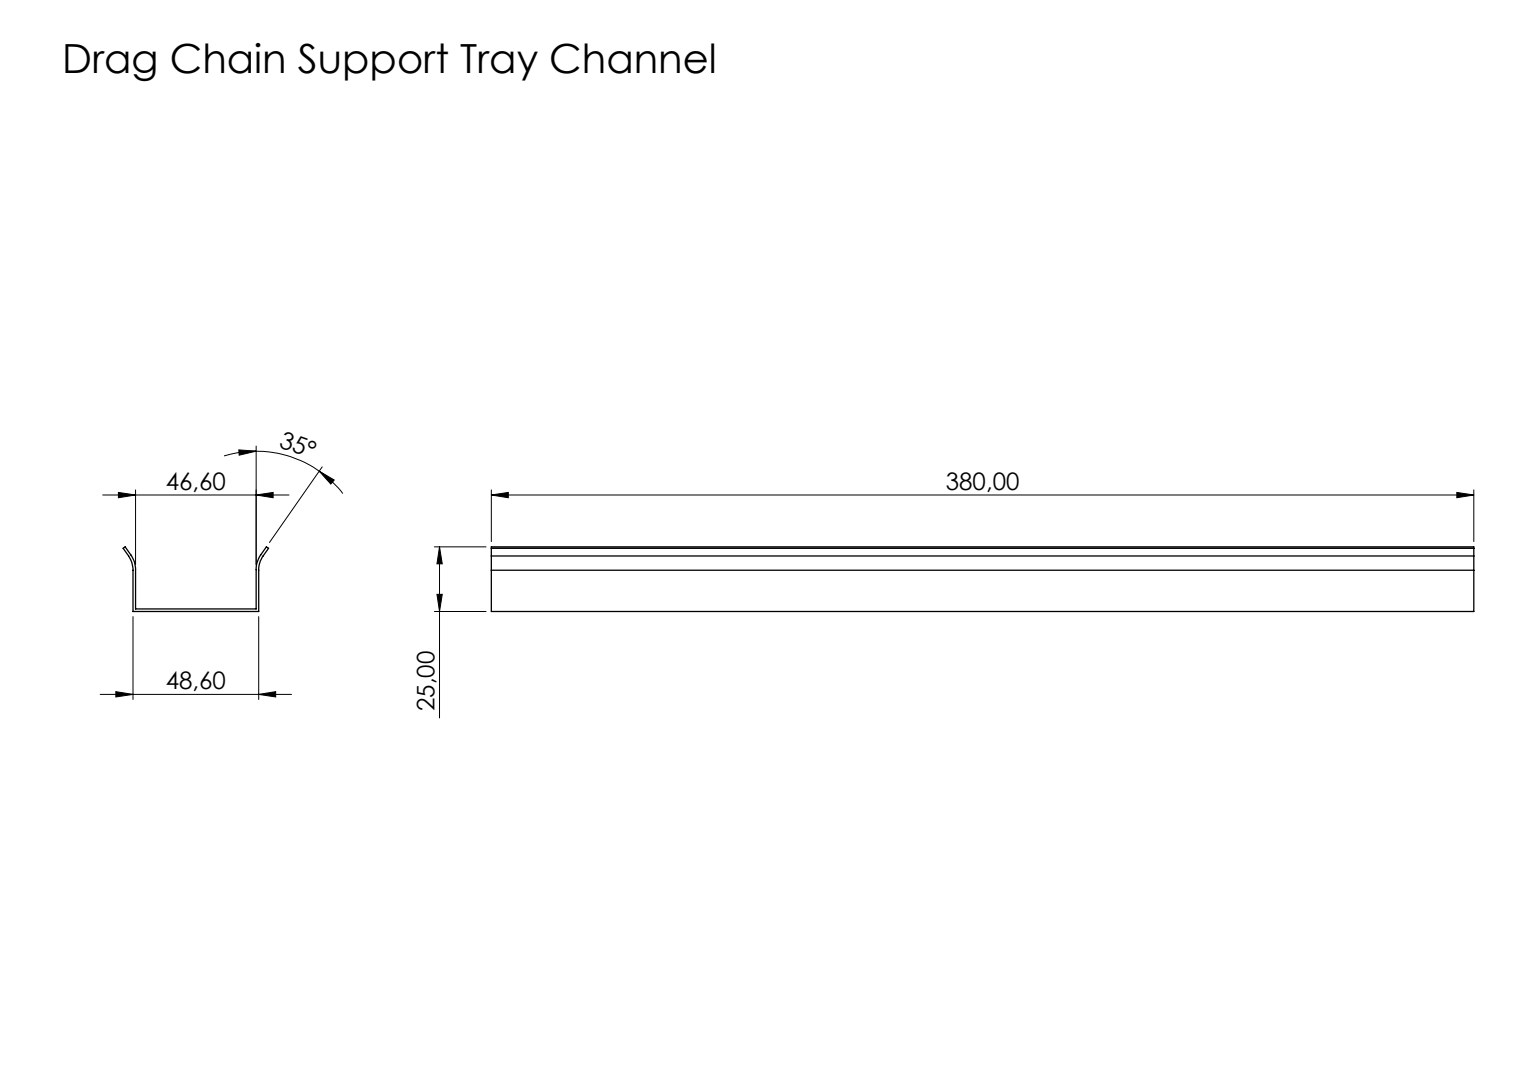
ISO-10303-21;
HEADER;
FILE_DESCRIPTION (('STEP AP214'),
    '1' );
FILE_NAME ('Drag Chain Support Tray Channel.step',
    '2026-10-08T22:59:04',
    ( '' ),
    ( '' ),
    'SwSTEP 2.0',
    'SolidWorks 2020',
    '' );
FILE_SCHEMA (( 'AUTOMOTIVE_DESIGN' ));
ENDSEC;

DATA;
#73=CARTESIAN_POINT ( 'NONE',  ( 33.30000000000001137, 3.332938107839120701, 33.00000000000000000 ) ) ;
#738=FACE_OUTER_BOUND ( 'NONE', #224116, .T. ) ;
#922=APPLICATION_CONTEXT ( 'automotive_design' ) ;
#1036=ORIENTED_EDGE ( 'NONE', *, *, #252988, .T. ) ;
#2425=AXIS2_PLACEMENT_3D ( 'NONE', #153513, #135160, #16531 ) ;
#2767=LINE ( 'NONE', #5320, #211110 ) ;
#3053=EDGE_CURVE ( 'NONE', #170483, #36666, #227559, .T. ) ;
#3540=CARTESIAN_POINT ( 'NONE',  ( 24.30000000000000071, 3.175288713399624818, -347.0000000000001137 ) ) ;
#4159=DIRECTION ( 'NONE',  ( 0.000000000000000000, 0.000000000000000000, 1.000000000000000000 ) ) ;
#4565=VECTOR ( 'NONE', #97094, 999.9999999999998863 ) ;
#4618=LINE ( 'NONE', #163716, #49347 ) ;
#4703=AXIS2_PLACEMENT_3D ( 'NONE', #177790, #57793, #79908 ) ;
#5320=CARTESIAN_POINT ( 'NONE',  ( 28.12018973533754362, 11.62642356364896123, 33.00000000000000000 ) ) ;
#5336=CIRCLE ( 'NONE', #192815, 9.500000000000001776 ) ;
#5403=ORIENTED_EDGE ( 'NONE', *, *, #105661, .F. ) ;
#5597=VERTEX_POINT ( 'NONE', #205200 ) ;
#5837=AXIS2_PLACEMENT_3D ( 'NONE', #3540, #257818, #144314 ) ;
#5882=LINE ( 'NONE', #127130, #156042 ) ;
#6762=EDGE_CURVE ( 'NONE', #161541, #211804, #135194, .T. ) ;
#6787=AXIS2_PLACEMENT_3D ( 'NONE', #52394, #130658, #31601 ) ;
#6946=ORIENTED_EDGE ( 'NONE', *, *, #257321, .T. ) ;
#7916=FACE_OUTER_BOUND ( 'NONE', #129895, .T. ) ;
#8087=ORIENTED_EDGE ( 'NONE', *, *, #57923, .T. ) ;
#8445=DIRECTION ( 'NONE',  ( 0.8191520442889919096, -0.5735764363510460484, 0.000000000000000000 ) ) ;
#9694=ORIENTED_EDGE ( 'NONE', *, *, #126812, .T. ) ;
#11133=DIRECTION ( 'NONE',  ( 1.000000000000000000, 0.000000000000000000, 0.000000000000000000 ) ) ;
#11208=ADVANCED_FACE ( 'NONE', ( #78803 ), #179241, .F. ) ;
#11741=AXIS2_PLACEMENT_3D ( 'NONE', #168935, #248426, #189738 ) ;
#13839=ADVANCED_BREP_SHAPE_REPRESENTATION ( '', ( #193773, #2425 ), #147622 ) ;
#14104=ORIENTED_EDGE ( 'NONE', *, *, #134158, .T. ) ;
#14595=PLANE ( 'NONE',  #6787 ) ;
#16293=CARTESIAN_POINT ( 'NONE',  ( 24.30000000000000071, -12.79999999999999716, -347.0000000000001137 ) ) ;
#16531=DIRECTION ( 'NONE',  ( 1.000000000000000000, 0.000000000000000000, 0.000000000000000000 ) ) ;
#16973=CARTESIAN_POINT ( 'NONE',  ( -27.30103769104855971, 12.19999999999999574, -347.0000000000001137 ) ) ;
#17586=CARTESIAN_POINT ( 'NONE',  ( -27.30103769104855971, 12.19999999999999574, 33.00000000000000000 ) ) ;
#17889=CARTESIAN_POINT ( 'NONE',  ( -24.30000000000000071, 3.175288713399619045, 33.00000000000000000 ) ) ;
#18117=DIRECTION ( 'NONE',  ( 0.5735764363510460484, -0.8191520442889919096, 0.000000000000000000 ) ) ;
#18168=DIRECTION ( 'NONE',  ( 1.070816960479510500E-16, -1.000000000000000000, 0.000000000000000000 ) ) ;
#18849=CARTESIAN_POINT ( 'NONE',  ( 33.30000000000001137, 3.332938107839120701, 33.00000000000000000 ) ) ;
#19405=ORIENTED_EDGE ( 'NONE', *, *, #195711, .T. ) ;
#19702=PLANE ( 'NONE',  #213240 ) ;
#19758=DIRECTION ( 'NONE',  ( -1.000000000000000000, 0.000000000000000000, 0.000000000000000000 ) ) ;
#20570=PLANE ( 'NONE',  #5837 ) ;
#20732=EDGE_LOOP ( 'NONE', ( #78906, #26119, #97741, #47134 ) ) ;
#20927=DIRECTION ( 'NONE',  ( -1.000000000000000000, 0.000000000000000000, 0.000000000000000000 ) ) ;
#21145=EDGE_CURVE ( 'NONE', #21183, #211804, #162402, .T. ) ;
#21183=VERTEX_POINT ( 'NONE', #80239 ) ;
#21763=ORIENTED_EDGE ( 'NONE', *, *, #207928, .T. ) ;
#21791=EDGE_CURVE ( 'NONE', #129045, #52293, #190662, .T. ) ;
#22213=VECTOR ( 'NONE', #257517, 1000.000000000000000 ) ;
#22259=CARTESIAN_POINT ( 'NONE',  ( 24.30000000000000071, 3.175288713399624818, 33.00000000000000000 ) ) ;
#22351=CARTESIAN_POINT ( 'NONE',  ( -24.30000000000000071, 3.175288713399619045, -347.0000000000001137 ) ) ;
#22631=LINE ( 'NONE', #102112, #93911 ) ;
#23564=ORIENTED_EDGE ( 'NONE', *, *, #151707, .T. ) ;
#23567=DIRECTION ( 'NONE',  ( -0.000000000000000000, 1.000000000000000000, -0.000000000000000000 ) ) ;
#23597=CARTESIAN_POINT ( 'NONE',  ( -33.80000000000000426, 3.175288713399618601, -347.0000000000001137 ) ) ;
#23706=( LENGTH_UNIT ( ) NAMED_UNIT ( * ) SI_UNIT ( .MILLI., .METRE. ) );
#24444=CLOSED_SHELL ( 'NONE', ( #93514, #231899, #33585, #223638, #74734, #90628, #232417, #255096, #257586, #97914, #165410, #200576, #127157, #116588, #142229, #84628, #136428, #11208 ) ) ;
#25351=EDGE_CURVE ( 'NONE', #161541, #81489, #168111, .T. ) ;
#25723=APPLICATION_CONTEXT ( 'automotive_design' ) ;
#26119=ORIENTED_EDGE ( 'NONE', *, *, #173029, .F. ) ;
#26230=VERTEX_POINT ( 'NONE', #239541 ) ;
#26815=( LENGTH_UNIT ( ) NAMED_UNIT ( * ) SI_UNIT ( .MILLI., .METRE. ) );
#26974=SHAPE_REPRESENTATION ( 'Drag Chain Support Tray Channel', ( #2425 ), #147622 ) ;
#27239=ORIENTED_EDGE ( 'NONE', *, *, #127036, .T. ) ;
#28179=ORIENTED_EDGE ( 'NONE', *, *, #162458, .F. ) ;
#28703=ORIENTED_EDGE ( 'NONE', *, *, #230771, .T. ) ;
#28742=VECTOR ( 'NONE', #138929, 1000.000000000000000 ) ;
#28860=VERTEX_POINT ( 'NONE', #101014 ) ;
#29155=ORIENTED_EDGE ( 'NONE', *, *, #182694, .T. ) ;
#29427=( GEOMETRIC_REPRESENTATION_CONTEXT ( 3 ) GLOBAL_UNCERTAINTY_ASSIGNED_CONTEXT ( ( #47787 ) ) GLOBAL_UNIT_ASSIGNED_CONTEXT ( ( #23706, #79762, #159350 ) ) REPRESENTATION_CONTEXT ( 'NONE', 'WORKASPACE' ) );
#29963=VECTOR ( 'NONE', #214620, 1000.000000000000000 ) ;
#30285=CARTESIAN_POINT ( 'NONE',  ( -24.30000000000000071, -12.80000000000000249, 33.00000000000000000 ) ) ;
#30300=ORIENTED_EDGE ( 'NONE', *, *, #3053, .T. ) ;
#30661=FILL_AREA_STYLE_COLOUR ( '', #135708 ) ;
#30927=ORIENTED_EDGE ( 'NONE', *, *, #130588, .T. ) ;
#31601=DIRECTION ( 'NONE',  ( -1.000000000000000000, -1.116774769942150098E-16, 0.000000000000000000 ) ) ;
#31615=ORIENTED_EDGE ( 'NONE', *, *, #154307, .F. ) ;
#31650=DIRECTION ( 'NONE',  ( -0.8191520442889914655, 0.5735764363510466035, 0.000000000000000000 ) ) ;
#32019=AXIS2_PLACEMENT_3D ( 'NONE', #73643, #131013, #153189 ) ;
#32279=CARTESIAN_POINT ( 'NONE',  ( 23.30000000000000426, 3.332938107839120701, 33.00000000000000000 ) ) ;
#32646=EDGE_CURVE ( 'NONE', #58739, #220374, #149831, .T. ) ;
#32834=ORIENTED_EDGE ( 'NONE', *, *, #151707, .F. ) ;
#33530=STYLED_ITEM ( 'NONE', ( #199767 ), #193773 ) ;
#33585=ADVANCED_FACE ( 'NONE', ( #196977 ), #256914, .T. ) ;
#34708=LINE ( 'NONE', #235434, #22213 ) ;
#34764=EDGE_CURVE ( 'NONE', #28860, #179923, #4618, .T. ) ;
#34785=DIRECTION ( 'NONE',  ( -0.000000000000000000, -0.000000000000000000, -1.000000000000000000 ) ) ;
#36258=ORIENTED_EDGE ( 'NONE', *, *, #252988, .F. ) ;
#36666=VERTEX_POINT ( 'NONE', #224393 ) ;
#36717=VECTOR ( 'NONE', #251880, 1000.000000000000000 ) ;
#37418=DIRECTION ( 'NONE',  ( 0.000000000000000000, 0.000000000000000000, 1.000000000000000000 ) ) ;
#38131=CARTESIAN_POINT ( 'NONE',  ( -24.30000000000000071, 3.175288713399619933, -347.0000000000001137 ) ) ;
#38192=EDGE_CURVE ( 'NONE', #81489, #129962, #210850, .T. ) ;
#39279=CARTESIAN_POINT ( 'NONE',  ( -27.30103769104855971, 12.19999999999999574, -347.0000000000001137 ) ) ;
#40331=DIRECTION ( 'NONE',  ( 0.000000000000000000, 0.000000000000000000, 1.000000000000000000 ) ) ;
#40973=VERTEX_POINT ( 'NONE', #97492 ) ;
#41222=VECTOR ( 'NONE', #168357, 999.9999999999998863 ) ;
#41767=LINE ( 'NONE', #121321, #217642 ) ;
#42076=VECTOR ( 'NONE', #167900, 1000.000000000000000 ) ;
#42249=VECTOR ( 'NONE', #96464, 1000.000000000000000 ) ;
#43561=CARTESIAN_POINT ( 'NONE',  ( -25.10847955711009760, 9.068702471349583405, 33.00000000000000000 ) ) ;
#44072=CARTESIAN_POINT ( 'NONE',  ( -27.30103769104855971, 12.19999999999999574, 33.00000000000000000 ) ) ;
#45239=DIRECTION ( 'NONE',  ( -0.5735764363510466035, 0.8191520442889914655, 0.000000000000000000 ) ) ;
#45827=DIRECTION ( 'NONE',  ( 0.000000000000000000, 1.000000000000000000, 0.000000000000000000 ) ) ;
#46873=VERTEX_POINT ( 'NONE', #193707 ) ;
#47134=ORIENTED_EDGE ( 'NONE', *, *, #188159, .T. ) ;
#47545=LINE ( 'NONE', #84070, #225389 ) ;
#47787=UNCERTAINTY_MEASURE_WITH_UNIT (LENGTH_MEASURE( 1.000000000000000082E-05 ), #23706, 'distance_accuracy_value', 'NONE');
#47845=ORIENTED_EDGE ( 'NONE', *, *, #137375, .T. ) ;
#48528=ORIENTED_EDGE ( 'NONE', *, *, #38192, .T. ) ;
#48882=EDGE_CURVE ( 'NONE', #26230, #237761, #200845, .T. ) ;
#49347=VECTOR ( 'NONE', #243231, 999.9999999999998863 ) ;
#49645=CARTESIAN_POINT ( 'NONE',  ( -23.30000000000000426, 3.332938107839114927, -347.0000000000001137 ) ) ;
#50043=CARTESIAN_POINT ( 'NONE',  ( -25.10847955711010115, 9.068702471349579852, -347.0000000000001137 ) ) ;
#50226=ORIENTED_EDGE ( 'NONE', *, *, #219810, .T. ) ;
#50978=ORIENTED_EDGE ( 'NONE', *, *, #229521, .T. ) ;
#51074=ORIENTED_EDGE ( 'NONE', *, *, #219810, .F. ) ;
#51411=AXIS2_PLACEMENT_3D ( 'NONE', #73, #234853, #56188 ) ;
#51578=DIRECTION ( 'NONE',  ( 0.000000000000000000, 0.000000000000000000, 1.000000000000000000 ) ) ;
#52293=VERTEX_POINT ( 'NONE', #196651 ) ;
#52394=CARTESIAN_POINT ( 'NONE',  ( -23.30000000000000426, -11.79999999999999893, -347.0000000000001137 ) ) ;
#54763=CARTESIAN_POINT ( 'NONE',  ( 25.10847955711010115, 9.068702471349586958, -347.0000000000001137 ) ) ;
#55259=VERTEX_POINT ( 'NONE', #121208 ) ;
#55531=ORIENTED_EDGE ( 'NONE', *, *, #137375, .F. ) ;
#55839=ORIENTED_EDGE ( 'NONE', *, *, #217458, .T. ) ;
#56188=DIRECTION ( 'NONE',  ( -1.000000000000000000, 0.000000000000000000, 0.000000000000000000 ) ) ;
#56286=DIRECTION ( 'NONE',  ( -0.5735764363510466035, 0.8191520442889914655, 0.000000000000000000 ) ) ;
#56926=VERTEX_POINT ( 'NONE', #44072 ) ;
#57427=VECTOR ( 'NONE', #93601, 1000.000000000000114 ) ;
#57793=DIRECTION ( 'NONE',  ( -1.000000000000000000, 0.000000000000000000, 0.000000000000000000 ) ) ;
#57923=EDGE_CURVE ( 'NONE', #204353, #55259, #22631, .T. ) ;
#58597=MECHANICAL_DESIGN_GEOMETRIC_PRESENTATION_REPRESENTATION('',(#33530),#29427);
#58739=VERTEX_POINT ( 'NONE', #250971 ) ;
#58939=VECTOR ( 'NONE', #161724, 999.9999999999998863 ) ;
#59421=DIRECTION ( 'NONE',  ( 1.000000000000000000, 0.000000000000000000, 0.000000000000000000 ) ) ;
#59987=EDGE_CURVE ( 'NONE', #237761, #40973, #47545, .T. ) ;
#61546=CARTESIAN_POINT ( 'NONE',  ( -23.30000000000000426, -11.79999999999999893, 33.00000000000000000 ) ) ;
#62381=ORIENTED_EDGE ( 'NONE', *, *, #195711, .F. ) ;
#62752=ORIENTED_EDGE ( 'NONE', *, *, #154307, .T. ) ;
#63510=FACE_OUTER_BOUND ( 'NONE', #20732, .T. ) ;
#63998=CARTESIAN_POINT ( 'NONE',  ( 26.01805557925458956, 8.624264858734573380, -347.0000000000001137 ) ) ;
#64397=CARTESIAN_POINT ( 'NONE',  ( -26.01805557925458956, 8.624264858734566275, -347.0000000000001137 ) ) ;
#64829=ORIENTED_EDGE ( 'NONE', *, *, #21145, .T. ) ;
#64851=ORIENTED_EDGE ( 'NONE', *, *, #68702, .F. ) ;
#65292=VECTOR ( 'NONE', #239977, 1000.000000000000000 ) ;
#65912=SURFACE_SIDE_STYLE ('',( #244534 ) ) ;
#66177=VERTEX_POINT ( 'NONE', #254523 ) ;
#67192=ORIENTED_EDGE ( 'NONE', *, *, #160251, .F. ) ;
#67734=CARTESIAN_POINT ( 'NONE',  ( 28.12018973533754362, 11.62642356364896123, 33.00000000000000000 ) ) ;
#68679=ORIENTED_EDGE ( 'NONE', *, *, #83916, .T. ) ;
#68702=EDGE_CURVE ( 'NONE', #179923, #21183, #208518, .T. ) ;
#69173=VECTOR ( 'NONE', #37418, 1000.000000000000000 ) ;
#69320=ORIENTED_EDGE ( 'NONE', *, *, #212823, .F. ) ;
#69783=( NAMED_UNIT ( * ) SI_UNIT ( $, .STERADIAN. ) SOLID_ANGLE_UNIT ( ) );
#70569=VECTOR ( 'NONE', #202671, 1000.000000000000000 ) ;
#70929=DIRECTION ( 'NONE',  ( -0.5735764363510466035, 0.8191520442889914655, 0.000000000000000000 ) ) ;
#70982=ORIENTED_EDGE ( 'NONE', *, *, #25351, .F. ) ;
#71071=CARTESIAN_POINT ( 'NONE',  ( -28.12018973533754362, 11.62642356364895413, -347.0000000000001137 ) ) ;
#71558=DIRECTION ( 'NONE',  ( -1.000000000000000000, 0.000000000000000000, 0.000000000000000000 ) ) ;
#72406=CARTESIAN_POINT ( 'NONE',  ( 33.30000000000001137, 3.332938107839120701, -347.0000000000001137 ) ) ;
#73214=ORIENTED_EDGE ( 'NONE', *, *, #113570, .T. ) ;
#73449=CARTESIAN_POINT ( 'NONE',  ( 33.80000000000000426, 3.175288713399626594, 33.00000000000000000 ) ) ;
#73643=CARTESIAN_POINT ( 'NONE',  ( -33.30000000000001137, 3.332938107839112263, 33.00000000000000000 ) ) ;
#74264=ORIENTED_EDGE ( 'NONE', *, *, #110996, .F. ) ;
#74498=FACE_OUTER_BOUND ( 'NONE', #240879, .T. ) ;
#74734=ADVANCED_FACE ( 'NONE', ( #74498 ), #91457, .F. ) ;
#75272=CARTESIAN_POINT ( 'NONE',  ( -26.01805557925458956, 8.624264858734566275, -347.0000000000001137 ) ) ;
#75769=LINE ( 'NONE', #155329, #158506 ) ;
#75867=CARTESIAN_POINT ( 'NONE',  ( -25.10847955711010115, 9.068702471349579852, 33.00000000000000000 ) ) ;
#76434=DIRECTION ( 'NONE',  ( 1.000000000000000000, 0.000000000000000000, 0.000000000000000000 ) ) ;
#76440=ORIENTED_EDGE ( 'NONE', *, *, #32646, .F. ) ;
#77362=PLANE ( 'NONE',  #4703 ) ;
#78653=AXIS2_PLACEMENT_3D ( 'NONE', #22351, #226943, #101830 ) ;
#78769=EDGE_CURVE ( 'NONE', #149519, #140456, #250374, .T. ) ;
#78803=FACE_OUTER_BOUND ( 'NONE', #97567, .T. ) ;
#78906=ORIENTED_EDGE ( 'NONE', *, *, #115777, .F. ) ;
#78993=CARTESIAN_POINT ( 'NONE',  ( -23.30000000000000426, -11.79999999999999893, -347.0000000000001137 ) ) ;
#79246=COLOUR_RGB ( '', 0.40784314, 0.44705882, 0.49803922) ;
#79483=ORIENTED_EDGE ( 'NONE', *, *, #230771, .F. ) ;
#79760=VECTOR ( 'NONE', #107601, 1000.000000000000000 ) ;
#79762=( NAMED_UNIT ( * ) PLANE_ANGLE_UNIT ( ) SI_UNIT ( $, .RADIAN. ) );
#79779=LINE ( 'NONE', #38131, #95152 ) ;
#79908=DIRECTION ( 'NONE',  ( 0.000000000000000000, 0.000000000000000000, 1.000000000000000000 ) ) ;
#79955=CARTESIAN_POINT ( 'NONE',  ( 28.12018973533754362, 11.62642356364896123, -347.0000000000001137 ) ) ;
#80239=CARTESIAN_POINT ( 'NONE',  ( -28.12018973533754362, 11.62642356364895413, 33.00000000000000000 ) ) ;
#80333=EDGE_CURVE ( 'NONE', #26230, #201551, #149749, .T. ) ;
#80686=DIRECTION ( 'NONE',  ( 1.000000000000000000, 1.070816960479510500E-16, 0.000000000000000000 ) ) ;
#81053=SURFACE_SIDE_STYLE ('',( #198454 ) ) ;
#81106=ORIENTED_EDGE ( 'NONE', *, *, #257321, .F. ) ;
#81489=VERTEX_POINT ( 'NONE', #178338 ) ;
#81772=DIRECTION ( 'NONE',  ( 1.000000000000000000, 0.000000000000000000, 0.000000000000000000 ) ) ;
#81834=CIRCLE ( 'NONE', #32019, 10.00000000000000178 ) ;
#81892=ORIENTED_EDGE ( 'NONE', *, *, #57923, .F. ) ;
#82192=DIRECTION ( 'NONE',  ( -0.5735764363510457153, 0.8191520442889921316, 0.000000000000000000 ) ) ;
#82669=ORIENTED_EDGE ( 'NONE', *, *, #105661, .T. ) ;
#82830=ORIENTED_EDGE ( 'NONE', *, *, #207928, .F. ) ;
#82887=EDGE_CURVE ( 'NONE', #46873, #28860, #204295, .T. ) ;
#83916=EDGE_CURVE ( 'NONE', #179923, #161541, #75769, .T. ) ;
#83918=DIRECTION ( 'NONE',  ( 0.000000000000000000, -1.000000000000000000, 0.000000000000000000 ) ) ;
#84070=CARTESIAN_POINT ( 'NONE',  ( 25.10847955711010115, 9.068702471349586958, 33.00000000000000000 ) ) ;
#84497=ORIENTED_EDGE ( 'NONE', *, *, #82887, .F. ) ;
#84628=ADVANCED_FACE ( 'NONE', ( #239025 ), #77362, .T. ) ;
#84772=DIRECTION ( 'NONE',  ( 1.000000000000000000, 0.000000000000000000, 0.000000000000000000 ) ) ;
#84811=LINE ( 'NONE', #226925, #245445 ) ;
#85432=FILL_AREA_STYLE ('',( #30661 ) ) ;
#86404=AXIS2_PLACEMENT_3D ( 'NONE', #72406, #151949, #11133 ) ;
#86655=DIRECTION ( 'NONE',  ( 0.5735764363510460484, 0.8191520442889919096, 0.000000000000000000 ) ) ;
#87564=VECTOR ( 'NONE', #45239, 1000.000000000000114 ) ;
#87971=ORIENTED_EDGE ( 'NONE', *, *, #109759, .F. ) ;
#89348=ORIENTED_EDGE ( 'NONE', *, *, #21791, .T. ) ;
#89356=AXIS2_PLACEMENT_3D ( 'NONE', #23597, #144759, #84772 ) ;
#90040=LINE ( 'NONE', #169641, #41222 ) ;
#90286=FACE_OUTER_BOUND ( 'NONE', #133485, .T. ) ;
#90628=ADVANCED_FACE ( 'NONE', ( #63510 ), #20570, .T. ) ;
#91036=VECTOR ( 'NONE', #56286, 1000.000000000000114 ) ;
#91457=CYLINDRICAL_SURFACE ( 'NONE', #216134, 9.500000000000001776 ) ;
#91898=DIRECTION ( 'NONE',  ( 0.000000000000000000, 0.000000000000000000, 1.000000000000000000 ) ) ;
#92510=DIRECTION ( 'NONE',  ( -0.8191520442889919096, -0.5735764363510460484, 0.000000000000000000 ) ) ;
#93514=ADVANCED_FACE ( 'NONE', ( #189765 ), #153242, .T. ) ;
#93601=DIRECTION ( 'NONE',  ( -0.5735764363510466035, -0.8191520442889914655, -0.000000000000000000 ) ) ;
#93911=VECTOR ( 'NONE', #162141, 1000.000000000000000 ) ;
#94227=VECTOR ( 'NONE', #205670, 1000.000000000000000 ) ;
#94230=EDGE_CURVE ( 'NONE', #149519, #26230, #90040, .T. ) ;
#95152=VECTOR ( 'NONE', #159363, 1000.000000000000000 ) ;
#95153=CARTESIAN_POINT ( 'NONE',  ( 28.12018973533754362, 11.62642356364896123, -347.0000000000001137 ) ) ;
#95300=DIRECTION ( 'NONE',  ( 1.000000000000000000, 0.000000000000000000, 0.000000000000000000 ) ) ;
#95442=ORIENTED_EDGE ( 'NONE', *, *, #153683, .T. ) ;
#96236=CARTESIAN_POINT ( 'NONE',  ( -28.12018973533754362, 11.62642356364895413, -347.0000000000001137 ) ) ;
#96464=DIRECTION ( 'NONE',  ( 0.000000000000000000, 0.000000000000000000, 1.000000000000000000 ) ) ;
#96655=VERTEX_POINT ( 'NONE', #226852 ) ;
#97094=DIRECTION ( 'NONE',  ( -0.8191520442889921316, -0.5735764363510457153, 0.000000000000000000 ) ) ;
#97204=ORIENTED_EDGE ( 'NONE', *, *, #130588, .F. ) ;
#97492=CARTESIAN_POINT ( 'NONE',  ( 25.10847955711010115, 9.068702471349586958, 33.00000000000000000 ) ) ;
#97567=EDGE_LOOP ( 'NONE', ( #14104, #62752, #21763, #174112, #82669, #232076, #29155, #64829, #50978, #50226, #89348, #248262, #19405, #28703, #95442, #166493 ) ) ;
#97741=ORIENTED_EDGE ( 'NONE', *, *, #183393, .T. ) ;
#97914=ADVANCED_FACE ( 'NONE', ( #233344 ), #196747, .T. ) ;
#98834=ORIENTED_EDGE ( 'NONE', *, *, #34764, .T. ) ;
#99151=CARTESIAN_POINT ( 'NONE',  ( 27.30103769104855971, 12.20000000000000284, -347.0000000000001137 ) ) ;
#100460=LINE ( 'NONE', #22259, #134339 ) ;
#101014=CARTESIAN_POINT ( 'NONE',  ( -27.30103769104855971, 12.19999999999999574, -347.0000000000001137 ) ) ;
#101100=DIRECTION ( 'NONE',  ( 0.000000000000000000, 0.000000000000000000, -1.000000000000000000 ) ) ;
#101111=DIRECTION ( 'NONE',  ( 0.000000000000000000, 0.000000000000000000, 1.000000000000000000 ) ) ;
#101339=ORIENTED_EDGE ( 'NONE', *, *, #94230, .F. ) ;
#101343=AXIS2_PLACEMENT_3D ( 'NONE', #78993, #59421, #101100 ) ;
#101830=DIRECTION ( 'NONE',  ( 0.000000000000000000, 0.000000000000000000, 1.000000000000000000 ) ) ;
#102112=CARTESIAN_POINT ( 'NONE',  ( -23.30000000000000426, 3.332938107839114927, -347.0000000000001137 ) ) ;
#102366=VECTOR ( 'NONE', #151104, 1000.000000000000000 ) ;
#102623=FACE_OUTER_BOUND ( 'NONE', #123811, .T. ) ;
#103902=CARTESIAN_POINT ( 'NONE',  ( -25.10847955711010115, 9.068702471349579852, -347.0000000000001137 ) ) ;
#104347=CYLINDRICAL_SURFACE ( 'NONE', #89356, 9.500000000000001776 ) ;
#105164=PRODUCT_DEFINITION_CONTEXT ( 'detailed design', #922, 'design' ) ;
#105371=ORIENTED_EDGE ( 'NONE', *, *, #32646, .T. ) ;
#105661=EDGE_CURVE ( 'NONE', #55259, #109463, #81834, .T. ) ;
#107058=AXIS2_PLACEMENT_3D ( 'NONE', #217912, #198373, #19758 ) ;
#107599=PRODUCT_DEFINITION_SHAPE ( 'NONE', 'NONE',  #222081 ) ;
#107601=DIRECTION ( 'NONE',  ( -0.000000000000000000, 1.000000000000000000, -0.000000000000000000 ) ) ;
#109463=VERTEX_POINT ( 'NONE', #43561 ) ;
#109759=EDGE_CURVE ( 'NONE', #81489, #173014, #79779, .T. ) ;
#110060=DIRECTION ( 'NONE',  ( -0.8191520442889921316, 0.5735764363510457153, 0.000000000000000000 ) ) ;
#110555=ORIENTED_EDGE ( 'NONE', *, *, #183393, .F. ) ;
#110996=EDGE_CURVE ( 'NONE', #109463, #56926, #233669, .T. ) ;
#111156=DIRECTION ( 'NONE',  ( -0.5735764363510466035, -0.8191520442889914655, 0.000000000000000000 ) ) ;
#111355=DIRECTION ( 'NONE',  ( 0.5735764363510457153, 0.8191520442889921316, -0.000000000000000000 ) ) ;
#112400=ORIENTED_EDGE ( 'NONE', *, *, #59987, .F. ) ;
#112922=UNCERTAINTY_MEASURE_WITH_UNIT (LENGTH_MEASURE( 1.000000000000000082E-05 ), #184562, 'distance_accuracy_value', 'NONE');
#113218=FACE_OUTER_BOUND ( 'NONE', #233022, .T. ) ;
#113570=EDGE_CURVE ( 'NONE', #28860, #56926, #195617, .T. ) ;
#113644=ORIENTED_EDGE ( 'NONE', *, *, #235689, .T. ) ;
#114332=AXIS2_PLACEMENT_3D ( 'NONE', #209764, #173251, #71558 ) ;
#115777=EDGE_CURVE ( 'NONE', #52293, #206485, #100460, .T. ) ;
#116588=ADVANCED_FACE ( 'NONE', ( #738 ), #238087, .T. ) ;
#117762=AXIS2_PLACEMENT_3D ( 'NONE', #173396, #92510, #18117 ) ;
#121208=CARTESIAN_POINT ( 'NONE',  ( -23.30000000000000426, 3.332938107839114927, 33.00000000000000000 ) ) ;
#121321=CARTESIAN_POINT ( 'NONE',  ( -23.30000000000000426, -11.79999999999999893, -347.0000000000001137 ) ) ;
#121324=DIRECTION ( 'NONE',  ( 0.000000000000000000, 0.000000000000000000, 1.000000000000000000 ) ) ;
#122075=ORIENTED_EDGE ( 'NONE', *, *, #82887, .T. ) ;
#122227=CYLINDRICAL_SURFACE ( 'NONE', #212105, 10.00000000000000178 ) ;
#122708=ORIENTED_EDGE ( 'NONE', *, *, #78769, .F. ) ;
#123150=LINE ( 'NONE', #143975, #70569 ) ;
#123811=EDGE_LOOP ( 'NONE', ( #5403, #81892, #47845, #27239 ) ) ;
#125209=EDGE_LOOP ( 'NONE', ( #250001, #64851, #68679, #185496 ) ) ;
#125806=PLANE ( 'NONE',  #211905 ) ;
#126812=EDGE_CURVE ( 'NONE', #170483, #149519, #183791, .T. ) ;
#127036=EDGE_CURVE ( 'NONE', #46873, #109463, #130217, .T. ) ;
#127113=CARTESIAN_POINT ( 'NONE',  ( 27.30103769104855971, 12.20000000000000284, 33.00000000000000000 ) ) ;
#127130=CARTESIAN_POINT ( 'NONE',  ( 25.10847955711010115, 9.068702471349586958, -347.0000000000001137 ) ) ;
#127157=ADVANCED_FACE ( 'NONE', ( #102623 ), #122227, .T. ) ;
#128486=ORIENTED_EDGE ( 'NONE', *, *, #83916, .F. ) ;
#129045=VERTEX_POINT ( 'NONE', #30285 ) ;
#129216=CARTESIAN_POINT ( 'NONE',  ( -23.30000000000000426, -11.79999999999999893, 33.00000000000000000 ) ) ;
#129663=ORIENTED_EDGE ( 'NONE', *, *, #3053, .F. ) ;
#129895=EDGE_LOOP ( 'NONE', ( #51074, #87971, #48528, #216376 ) ) ;
#129962=VERTEX_POINT ( 'NONE', #254748 ) ;
#130217=LINE ( 'NONE', #139188, #183069 ) ;
#130588=EDGE_CURVE ( 'NONE', #129962, #233085, #84811, .T. ) ;
#130658=DIRECTION ( 'NONE',  ( -1.116774769942150098E-16, 1.000000000000000000, 0.000000000000000000 ) ) ;
#131013=DIRECTION ( 'NONE',  ( 0.000000000000000000, 0.000000000000000000, 1.000000000000000000 ) ) ;
#131930=AXIS2_PLACEMENT_3D ( 'NONE', #50043, #249548, #70929 ) ;
#132297=SHAPE_REPRESENTATION_RELATIONSHIP ( 'NONE' , 'NONE' ,  #26974, #13839 ) ;
#132443=ORIENTED_EDGE ( 'NONE', *, *, #127036, .F. ) ;
#133485=EDGE_LOOP ( 'NONE', ( #112400, #230876, #186880, #6946 ) ) ;
#134158=EDGE_CURVE ( 'NONE', #40973, #209179, #218012, .T. ) ;
#134339=VECTOR ( 'NONE', #23567, 1000.000000000000000 ) ;
#135160=DIRECTION ( 'NONE',  ( 0.000000000000000000, 0.000000000000000000, 1.000000000000000000 ) ) ;
#135194=LINE ( 'NONE', #75272, #69173 ) ;
#135271=CARTESIAN_POINT ( 'NONE',  ( 23.30000000000000426, -11.79999999999999538, 33.00000000000000000 ) ) ;
#135530=CARTESIAN_POINT ( 'NONE',  ( 24.30000000000000071, -12.79999999999999716, -347.0000000000001137 ) ) ;
#135598=SHAPE_DEFINITION_REPRESENTATION ( #107599, #26974 ) ;
#135708=COLOUR_RGB ( '', 0.40784314, 0.44705882, 0.49803922) ;
#135779=VECTOR ( 'NONE', #83918, 1000.000000000000000 ) ;
#136254=CIRCLE ( 'NONE', #107058, 9.500000000000001776 ) ;
#136428=ADVANCED_FACE ( 'NONE', ( #113218 ), #252717, .T. ) ;
#137014=DIRECTION ( 'NONE',  ( 0.5735764363510460484, -0.8191520442889919096, 0.000000000000000000 ) ) ;
#137375=EDGE_CURVE ( 'NONE', #204353, #46873, #156441, .T. ) ;
#138254=CARTESIAN_POINT ( 'NONE',  ( -33.30000000000001137, 3.332938107839112263, -347.0000000000001137 ) ) ;
#138455=FILL_AREA_STYLE ('',( #242707 ) ) ;
#138929=DIRECTION ( 'NONE',  ( 0.5735764363510460484, -0.8191520442889919096, 0.000000000000000000 ) ) ;
#139188=CARTESIAN_POINT ( 'NONE',  ( -25.10847955711009760, 9.068702471349583405, -347.0000000000001137 ) ) ;
#139371=VECTOR ( 'NONE', #45827, 1000.000000000000000 ) ;
#139814=AXIS2_PLACEMENT_3D ( 'NONE', #138254, #121324, #20927 ) ;
#139999=CIRCLE ( 'NONE', #156814, 9.500000000000001776 ) ;
#140456=VERTEX_POINT ( 'NONE', #67734 ) ;
#142229=ADVANCED_FACE ( 'NONE', ( #232356 ), #14595, .T. ) ;
#143975=CARTESIAN_POINT ( 'NONE',  ( 23.30000000000000426, -11.79999999999999538, -347.0000000000001137 ) ) ;
#144314=DIRECTION ( 'NONE',  ( -0.000000000000000000, 0.000000000000000000, -1.000000000000000000 ) ) ;
#144759=DIRECTION ( 'NONE',  ( 0.000000000000000000, 0.000000000000000000, 1.000000000000000000 ) ) ;
#145432=SURFACE_STYLE_USAGE ( .BOTH. , #65912 ) ;
#146666=DIRECTION ( 'NONE',  ( 0.000000000000000000, 0.000000000000000000, 1.000000000000000000 ) ) ;
#146700=( NAMED_UNIT ( * ) PLANE_ANGLE_UNIT ( ) SI_UNIT ( $, .RADIAN. ) );
#147146=VECTOR ( 'NONE', #190424, 1000.000000000000000 ) ;
#147169=PRODUCT ( 'Drag Chain Support Tray Channel', 'Drag Chain Support Tray Channel', '', ( #155213 ) ) ;
#147622=( GEOMETRIC_REPRESENTATION_CONTEXT ( 3 ) GLOBAL_UNCERTAINTY_ASSIGNED_CONTEXT ( ( #112922 ) ) GLOBAL_UNIT_ASSIGNED_CONTEXT ( ( #184562, #146700, #69783 ) ) REPRESENTATION_CONTEXT ( 'NONE', 'WORKASPACE' ) );
#148220=ORIENTED_EDGE ( 'NONE', *, *, #109759, .T. ) ;
#149519=VERTEX_POINT ( 'NONE', #79955 ) ;
#149749=LINE ( 'NONE', #192708, #57427 ) ;
#149831=LINE ( 'NONE', #188944, #102366 ) ;
#150162=CARTESIAN_POINT ( 'NONE',  ( 33.80000000000000426, 3.175288713399626594, -347.0000000000001137 ) ) ;
#151104=DIRECTION ( 'NONE',  ( 0.000000000000000000, 0.000000000000000000, 1.000000000000000000 ) ) ;
#151594=CARTESIAN_POINT ( 'NONE',  ( 25.10847955711010115, 9.068702471349586958, -347.0000000000001137 ) ) ;
#151707=EDGE_CURVE ( 'NONE', #96655, #5597, #123150, .T. ) ;
#151949=DIRECTION ( 'NONE',  ( 0.000000000000000000, 0.000000000000000000, 1.000000000000000000 ) ) ;
#152877=ORIENTED_EDGE ( 'NONE', *, *, #199032, .F. ) ;
#153189=DIRECTION ( 'NONE',  ( -1.000000000000000000, 0.000000000000000000, 0.000000000000000000 ) ) ;
#153191=( NAMED_UNIT ( * ) PLANE_ANGLE_UNIT ( ) SI_UNIT ( $, .RADIAN. ) );
#153242=CYLINDRICAL_SURFACE ( 'NONE', #86404, 10.00000000000000178 ) ;
#153375=EDGE_LOOP ( 'NONE', ( #211139, #122708, #256282, #155091 ) ) ;
#153513=CARTESIAN_POINT ( 'NONE',  ( 0.000000000000000000, 0.000000000000000000, 0.000000000000000000 ) ) ;
#153683=EDGE_CURVE ( 'NONE', #140456, #237761, #203400, .T. ) ;
#154307=EDGE_CURVE ( 'NONE', #209179, #182327, #254973, .T. ) ;
#155091=ORIENTED_EDGE ( 'NONE', *, *, #48882, .T. ) ;
#155213=PRODUCT_CONTEXT ( 'NONE', #25723, 'mechanical' ) ;
#155329=CARTESIAN_POINT ( 'NONE',  ( -28.12018973533754362, 11.62642356364895413, -347.0000000000001137 ) ) ;
#155627=AXIS2_PLACEMENT_3D ( 'NONE', #239615, #163927, #238314 ) ;
#156042=VECTOR ( 'NONE', #146666, 1000.000000000000000 ) ;
#156245=DIRECTION ( 'NONE',  ( 0.000000000000000000, 0.000000000000000000, 1.000000000000000000 ) ) ;
#156441=CIRCLE ( 'NONE', #139814, 10.00000000000000178 ) ;
#156814=AXIS2_PLACEMENT_3D ( 'NONE', #213374, #34785, #76434 ) ;
#157102=DIRECTION ( 'NONE',  ( -1.000000000000000000, 0.000000000000000000, 0.000000000000000000 ) ) ;
#157251=EDGE_LOOP ( 'NONE', ( #31615, #239706, #23564, #255593 ) ) ;
#158363=EDGE_LOOP ( 'NONE', ( #79483, #129663, #9694, #229195 ) ) ;
#158506=VECTOR ( 'NONE', #137014, 1000.000000000000000 ) ;
#159350=( NAMED_UNIT ( * ) SI_UNIT ( $, .STERADIAN. ) SOLID_ANGLE_UNIT ( ) );
#159363=DIRECTION ( 'NONE',  ( 0.000000000000000000, 0.000000000000000000, 1.000000000000000000 ) ) ;
#160251=EDGE_CURVE ( 'NONE', #201551, #96655, #236555, .T. ) ;
#160459=CARTESIAN_POINT ( 'NONE',  ( 27.30103769104855971, 12.20000000000000284, -347.0000000000001137 ) ) ;
#160515=ORIENTED_EDGE ( 'NONE', *, *, #188159, .F. ) ;
#160645=SURFACE_STYLE_USAGE ( .BOTH. , #81053 ) ;
#161541=VERTEX_POINT ( 'NONE', #64397 ) ;
#161724=DIRECTION ( 'NONE',  ( -0.8191520442889921316, 0.5735764363510457153, -0.000000000000000000 ) ) ;
#161790=DIRECTION ( 'NONE',  ( -0.8191520442889921316, -0.5735764363510457153, 0.000000000000000000 ) ) ;
#161947=LINE ( 'NONE', #61546, #139371 ) ;
#162141=DIRECTION ( 'NONE',  ( 0.000000000000000000, 0.000000000000000000, 1.000000000000000000 ) ) ;
#162330=VECTOR ( 'NONE', #238317, 1000.000000000000000 ) ;
#162358=CARTESIAN_POINT ( 'NONE',  ( 23.30000000000000426, -11.79999999999999538, -347.0000000000001137 ) ) ;
#162402=LINE ( 'NONE', #176833, #28742 ) ;
#162458=EDGE_CURVE ( 'NONE', #129962, #129045, #228361, .T. ) ;
#163716=CARTESIAN_POINT ( 'NONE',  ( -27.30103769104855971, 12.19999999999999574, -347.0000000000001137 ) ) ;
#163927=DIRECTION ( 'NONE',  ( -0.000000000000000000, -0.000000000000000000, -1.000000000000000000 ) ) ;
#164386=MECHANICAL_DESIGN_GEOMETRIC_PRESENTATION_REPRESENTATION('',(#180948),#176868);
#165410=ADVANCED_FACE ( 'NONE', ( #237451 ), #19702, .T. ) ;
#165495=PRODUCT_DEFINITION_FORMATION_WITH_SPECIFIED_SOURCE ( 'ANY', '', #147169, .NOT_KNOWN. ) ;
#165524=DIRECTION ( 'NONE',  ( 0.5735764363510460484, 0.8191520442889919096, -0.000000000000000000 ) ) ;
#165679=VECTOR ( 'NONE', #181908, 1000.000000000000000 ) ;
#166269=DIRECTION ( 'NONE',  ( -0.5735764363510466035, -0.8191520442889914655, -0.000000000000000000 ) ) ;
#166493=ORIENTED_EDGE ( 'NONE', *, *, #59987, .T. ) ;
#166510=CARTESIAN_POINT ( 'NONE',  ( -33.30000000000001137, 3.332938107839112263, -347.0000000000001137 ) ) ;
#167900=DIRECTION ( 'NONE',  ( 0.000000000000000000, -1.000000000000000000, 0.000000000000000000 ) ) ;
#168111=CIRCLE ( 'NONE', #155627, 9.500000000000001776 ) ;
#168126=CARTESIAN_POINT ( 'NONE',  ( 28.12018973533754362, 11.62642356364896123, -347.0000000000001137 ) ) ;
#168357=DIRECTION ( 'NONE',  ( -0.8191520442889921316, 0.5735764363510457153, -0.000000000000000000 ) ) ;
#168564=ORIENTED_EDGE ( 'NONE', *, *, #235689, .F. ) ;
#168935=CARTESIAN_POINT ( 'NONE',  ( 33.30000000000001137, 3.332938107839120701, -347.0000000000001137 ) ) ;
#169641=CARTESIAN_POINT ( 'NONE',  ( 27.30103769104855971, 12.20000000000000284, -347.0000000000001137 ) ) ;
#170330=LINE ( 'NONE', #205536, #215033 ) ;
#170483=VERTEX_POINT ( 'NONE', #63998 ) ;
#171621=EDGE_LOOP ( 'NONE', ( #82830, #69320, #1036, #105371 ) ) ;
#171752=CARTESIAN_POINT ( 'NONE',  ( -24.30000000000000071, 3.175288713399619045, -347.0000000000001137 ) ) ;
#172457=PLANE ( 'NONE',  #182628 ) ;
#172778=ORIENTED_EDGE ( 'NONE', *, *, #25351, .T. ) ;
#172875=LINE ( 'NONE', #17586, #4565 ) ;
#172939=UNCERTAINTY_MEASURE_WITH_UNIT (LENGTH_MEASURE( 1.000000000000000082E-05 ), #26815, 'distance_accuracy_value', 'NONE');
#173014=VERTEX_POINT ( 'NONE', #239779 ) ;
#173029=EDGE_CURVE ( 'NONE', #233085, #52293, #177263, .T. ) ;
#173251=DIRECTION ( 'NONE',  ( -0.000000000000000000, 0.000000000000000000, -1.000000000000000000 ) ) ;
#173396=CARTESIAN_POINT ( 'NONE',  ( -28.12018973533754362, 11.62642356364895413, -347.0000000000001137 ) ) ;
#173695=CARTESIAN_POINT ( 'NONE',  ( 24.30000000000000071, -12.79999999999999716, 33.00000000000000000 ) ) ;
#174112=ORIENTED_EDGE ( 'NONE', *, *, #199032, .T. ) ;
#175975=CARTESIAN_POINT ( 'NONE',  ( 24.30000000000000071, -12.79999999999999716, -347.0000000000001137 ) ) ;
#175985=PLANE ( 'NONE',  #224482 ) ;
#176120=ORIENTED_EDGE ( 'NONE', *, *, #113570, .F. ) ;
#176693=CARTESIAN_POINT ( 'NONE',  ( -26.01805557925458956, 8.624264858734566275, 33.00000000000000000 ) ) ;
#176833=CARTESIAN_POINT ( 'NONE',  ( -28.12018973533754362, 11.62642356364895413, 33.00000000000000000 ) ) ;
#176868=( GEOMETRIC_REPRESENTATION_CONTEXT ( 3 ) GLOBAL_UNCERTAINTY_ASSIGNED_CONTEXT ( ( #172939 ) ) GLOBAL_UNIT_ASSIGNED_CONTEXT ( ( #26815, #153191, #233966 ) ) REPRESENTATION_CONTEXT ( 'NONE', 'WORKASPACE' ) );
#177263=LINE ( 'NONE', #175975, #210834 ) ;
#177433=ORIENTED_EDGE ( 'NONE', *, *, #126812, .F. ) ;
#177499=ORIENTED_EDGE ( 'NONE', *, *, #21791, .F. ) ;
#177790=CARTESIAN_POINT ( 'NONE',  ( 23.30000000000000426, -11.79999999999999538, -347.0000000000001137 ) ) ;
#178338=CARTESIAN_POINT ( 'NONE',  ( -24.30000000000000071, 3.175288713399619933, -347.0000000000001137 ) ) ;
#179241=PLANE ( 'NONE',  #242650 ) ;
#179923=VERTEX_POINT ( 'NONE', #71071 ) ;
#180948=STYLED_ITEM ( 'NONE', ( #224958 ), #13839 ) ;
#181908=DIRECTION ( 'NONE',  ( 0.000000000000000000, 0.000000000000000000, 1.000000000000000000 ) ) ;
#182327=VERTEX_POINT ( 'NONE', #135271 ) ;
#182628=AXIS2_PLACEMENT_3D ( 'NONE', #151594, #31650, #111156 ) ;
#182694=EDGE_CURVE ( 'NONE', #56926, #21183, #172875, .T. ) ;
#182835=CARTESIAN_POINT ( 'NONE',  ( -24.30000000000000071, -12.80000000000000249, -347.0000000000001137 ) ) ;
#183069=VECTOR ( 'NONE', #156245, 1000.000000000000000 ) ;
#183393=EDGE_CURVE ( 'NONE', #233085, #66177, #223684, .T. ) ;
#183791=LINE ( 'NONE', #168126, #240473 ) ;
#184562=( LENGTH_UNIT ( ) NAMED_UNIT ( * ) SI_UNIT ( .MILLI., .METRE. ) );
#185253=PLANE ( 'NONE',  #78653 ) ;
#185496=ORIENTED_EDGE ( 'NONE', *, *, #6762, .T. ) ;
#185842=CARTESIAN_POINT ( 'NONE',  ( 23.30000000000000426, 3.332938107839120701, -347.0000000000001137 ) ) ;
#185857=CARTESIAN_POINT ( 'NONE',  ( 24.30000000000000071, 3.175288713399624818, -347.0000000000001137 ) ) ;
#186170=AXIS2_PLACEMENT_3D ( 'NONE', #99151, #111355, #110060 ) ;
#186880=ORIENTED_EDGE ( 'NONE', *, *, #80333, .T. ) ;
#188159=EDGE_CURVE ( 'NONE', #66177, #206485, #170330, .T. ) ;
#188684=CARTESIAN_POINT ( 'NONE',  ( -23.30000000000000426, -11.79999999999999893, -347.0000000000001137 ) ) ;
#188936=ORIENTED_EDGE ( 'NONE', *, *, #182694, .F. ) ;
#188944=CARTESIAN_POINT ( 'NONE',  ( -23.30000000000000426, -11.79999999999999893, -347.0000000000001137 ) ) ;
#189738=DIRECTION ( 'NONE',  ( -1.000000000000000000, 0.000000000000000000, 0.000000000000000000 ) ) ;
#189765=FACE_OUTER_BOUND ( 'NONE', #196024, .T. ) ;
#190424=DIRECTION ( 'NONE',  ( 0.000000000000000000, 0.000000000000000000, 1.000000000000000000 ) ) ;
#190662=LINE ( 'NONE', #173695, #36717 ) ;
#190878=PLANE ( 'NONE',  #131930 ) ;
#191997=ORIENTED_EDGE ( 'NONE', *, *, #253132, .F. ) ;
#192708=CARTESIAN_POINT ( 'NONE',  ( 25.10847955711010115, 9.068702471349586958, -347.0000000000001137 ) ) ;
#192815=AXIS2_PLACEMENT_3D ( 'NONE', #73449, #212932, #233789 ) ;
#193707=CARTESIAN_POINT ( 'NONE',  ( -25.10847955711009760, 9.068702471349583405, -347.0000000000001137 ) ) ;
#193773=MANIFOLD_SOLID_BREP ( 'Stock-MAS-200-1', #24444 ) ;
#194425=DIRECTION ( 'NONE',  ( 0.000000000000000000, 0.000000000000000000, 1.000000000000000000 ) ) ;
#195617=LINE ( 'NONE', #16973, #42249 ) ;
#195711=EDGE_CURVE ( 'NONE', #206485, #36666, #5336, .T. ) ;
#196024=EDGE_LOOP ( 'NONE', ( #207658, #81106, #211538, #55839 ) ) ;
#196651=CARTESIAN_POINT ( 'NONE',  ( 24.30000000000000071, -12.79999999999999716, 33.00000000000000000 ) ) ;
#196747=PLANE ( 'NONE',  #117762 ) ;
#196794=FACE_OUTER_BOUND ( 'NONE', #220903, .T. ) ;
#196977=FACE_OUTER_BOUND ( 'NONE', #153375, .T. ) ;
#197626=CARTESIAN_POINT ( 'NONE',  ( 23.30000000000000426, -11.79999999999999538, 33.00000000000000000 ) ) ;
#198373=DIRECTION ( 'NONE',  ( -0.000000000000000000, -0.000000000000000000, -1.000000000000000000 ) ) ;
#198454=SURFACE_STYLE_FILL_AREA ( #138455 ) ;
#199032=EDGE_CURVE ( 'NONE', #220374, #55259, #161947, .T. ) ;
#199767=PRESENTATION_STYLE_ASSIGNMENT (( #160645 ) ) ;
#200276=LINE ( 'NONE', #185842, #255832 ) ;
#200576=ADVANCED_FACE ( 'NONE', ( #228704 ), #190878, .T. ) ;
#200821=DIRECTION ( 'NONE',  ( 0.000000000000000000, 1.000000000000000000, 0.000000000000000000 ) ) ;
#200845=LINE ( 'NONE', #160459, #65292 ) ;
#201551=VERTEX_POINT ( 'NONE', #54763 ) ;
#202276=DIRECTION ( 'NONE',  ( 0.5735764363510460484, 0.8191520442889919096, -0.000000000000000000 ) ) ;
#202671=DIRECTION ( 'NONE',  ( -0.000000000000000000, -1.000000000000000000, -0.000000000000000000 ) ) ;
#203029=DIRECTION ( 'NONE',  ( 0.000000000000000000, 0.000000000000000000, 1.000000000000000000 ) ) ;
#203400=LINE ( 'NONE', #205956, #58939 ) ;
#204295=LINE ( 'NONE', #103902, #87564 ) ;
#204353=VERTEX_POINT ( 'NONE', #49645 ) ;
#204453=ORIENTED_EDGE ( 'NONE', *, *, #38192, .F. ) ;
#205200=CARTESIAN_POINT ( 'NONE',  ( 23.30000000000000426, -11.79999999999999538, -347.0000000000001137 ) ) ;
#205329=CARTESIAN_POINT ( 'NONE',  ( 28.12018973533754362, 11.62642356364896123, -347.0000000000001137 ) ) ;
#205536=CARTESIAN_POINT ( 'NONE',  ( 24.30000000000000071, 3.175288713399624818, -347.0000000000001137 ) ) ;
#205670=DIRECTION ( 'NONE',  ( -1.000000000000000000, -1.116774769942150098E-16, -0.000000000000000000 ) ) ;
#205956=CARTESIAN_POINT ( 'NONE',  ( 27.30103769104855971, 12.20000000000000284, 33.00000000000000000 ) ) ;
#206485=VERTEX_POINT ( 'NONE', #254890 ) ;
#207658=ORIENTED_EDGE ( 'NONE', *, *, #134158, .F. ) ;
#207928=EDGE_CURVE ( 'NONE', #182327, #220374, #34708, .T. ) ;
#208518=LINE ( 'NONE', #96236, #162330 ) ;
#209179=VERTEX_POINT ( 'NONE', #32279 ) ;
#209221=EDGE_LOOP ( 'NONE', ( #74264, #132443, #122075, #73214 ) ) ;
#209764=CARTESIAN_POINT ( 'NONE',  ( 33.30000000000001137, 3.332938107839120701, -347.0000000000001137 ) ) ;
#210187=ORIENTED_EDGE ( 'NONE', *, *, #68702, .T. ) ;
#210497=FACE_OUTER_BOUND ( 'NONE', #158363, .T. ) ;
#210834=VECTOR ( 'NONE', #40331, 1000.000000000000000 ) ;
#210850=LINE ( 'NONE', #171752, #42076 ) ;
#211110=VECTOR ( 'NONE', #202276, 1000.000000000000000 ) ;
#211139=ORIENTED_EDGE ( 'NONE', *, *, #153683, .F. ) ;
#211538=ORIENTED_EDGE ( 'NONE', *, *, #160251, .T. ) ;
#211582=ORIENTED_EDGE ( 'NONE', *, *, #80333, .F. ) ;
#211804=VERTEX_POINT ( 'NONE', #176693 ) ;
#211905=AXIS2_PLACEMENT_3D ( 'NONE', #205329, #8445, #86655 ) ;
#211988=VECTOR ( 'NONE', #4159, 1000.000000000000000 ) ;
#212105=AXIS2_PLACEMENT_3D ( 'NONE', #166510, #203029, #81772 ) ;
#212823=EDGE_CURVE ( 'NONE', #5597, #182327, #218438, .T. ) ;
#212932=DIRECTION ( 'NONE',  ( -0.000000000000000000, -0.000000000000000000, -1.000000000000000000 ) ) ;
#213240=AXIS2_PLACEMENT_3D ( 'NONE', #39279, #82192, #161790 ) ;
#213374=CARTESIAN_POINT ( 'NONE',  ( 33.80000000000000426, 3.175288713399626594, -347.0000000000001137 ) ) ;
#213907=ORIENTED_EDGE ( 'NONE', *, *, #173029, .T. ) ;
#214620=DIRECTION ( 'NONE',  ( -0.000000000000000000, -1.000000000000000000, -0.000000000000000000 ) ) ;
#215033=VECTOR ( 'NONE', #51578, 1000.000000000000000 ) ;
#216088=LINE ( 'NONE', #17889, #135779 ) ;
#216134=AXIS2_PLACEMENT_3D ( 'NONE', #150162, #194425, #95300 ) ;
#216376=ORIENTED_EDGE ( 'NONE', *, *, #162458, .T. ) ;
#217458=EDGE_CURVE ( 'NONE', #96655, #209179, #200276, .T. ) ;
#217642=VECTOR ( 'NONE', #200821, 1000.000000000000000 ) ;
#217912=CARTESIAN_POINT ( 'NONE',  ( -33.80000000000000426, 3.175288713399618601, 33.00000000000000000 ) ) ;
#218012=CIRCLE ( 'NONE', #51411, 10.00000000000000178 ) ;
#218438=LINE ( 'NONE', #162358, #165679 ) ;
#219810=EDGE_CURVE ( 'NONE', #173014, #129045, #216088, .T. ) ;
#220374=VERTEX_POINT ( 'NONE', #129216 ) ;
#220903=EDGE_LOOP ( 'NONE', ( #177499, #28179, #30927, #213907 ) ) ;
#221725=FACE_OUTER_BOUND ( 'NONE', #232385, .T. ) ;
#222081=PRODUCT_DEFINITION ( 'UNKNOWN', '', #165495, #105164 ) ;
#223066=DIRECTION ( 'NONE',  ( 1.000000000000000000, 1.070816960479510500E-16, -0.000000000000000000 ) ) ;
#223638=ADVANCED_FACE ( 'NONE', ( #210497 ), #125806, .T. ) ;
#223684=LINE ( 'NONE', #185857, #79760 ) ;
#224116=EDGE_LOOP ( 'NONE', ( #152877, #76440, #113644, #8087 ) ) ;
#224393=CARTESIAN_POINT ( 'NONE',  ( 26.01805557925458956, 8.624264858734573380, 33.00000000000000000 ) ) ;
#224482=AXIS2_PLACEMENT_3D ( 'NONE', #135530, #18168, #80686 ) ;
#224958=PRESENTATION_STYLE_ASSIGNMENT (( #145432 ) ) ;
#225222=LINE ( 'NONE', #188684, #94227 ) ;
#225389=VECTOR ( 'NONE', #166269, 1000.000000000000114 ) ;
#226852=CARTESIAN_POINT ( 'NONE',  ( 23.30000000000000426, 3.332938107839120701, -347.0000000000001137 ) ) ;
#226925=CARTESIAN_POINT ( 'NONE',  ( 24.30000000000000071, -12.79999999999999716, -347.0000000000001137 ) ) ;
#226943=DIRECTION ( 'NONE',  ( -1.000000000000000000, 0.000000000000000000, 0.000000000000000000 ) ) ;
#227559=LINE ( 'NONE', #232719, #230947 ) ;
#228361=LINE ( 'NONE', #182835, #211988 ) ;
#228704=FACE_OUTER_BOUND ( 'NONE', #209221, .T. ) ;
#229195=ORIENTED_EDGE ( 'NONE', *, *, #78769, .T. ) ;
#229521=EDGE_CURVE ( 'NONE', #211804, #173014, #136254, .T. ) ;
#230771=EDGE_CURVE ( 'NONE', #36666, #140456, #2767, .T. ) ;
#230876=ORIENTED_EDGE ( 'NONE', *, *, #48882, .F. ) ;
#230947=VECTOR ( 'NONE', #91898, 1000.000000000000000 ) ;
#231386=EDGE_LOOP ( 'NONE', ( #188936, #176120, #98834, #210187 ) ) ;
#231899=ADVANCED_FACE ( 'NONE', ( #90286 ), #172457, .T. ) ;
#232076=ORIENTED_EDGE ( 'NONE', *, *, #110996, .T. ) ;
#232356=FACE_OUTER_BOUND ( 'NONE', #171621, .T. ) ;
#232385=EDGE_LOOP ( 'NONE', ( #247353, #252060, #172778, #148220 ) ) ;
#232417=ADVANCED_FACE ( 'NONE', ( #196794 ), #175985, .T. ) ;
#232719=CARTESIAN_POINT ( 'NONE',  ( 26.01805557925458956, 8.624264858734573380, -347.0000000000001137 ) ) ;
#233022=EDGE_LOOP ( 'NONE', ( #67192, #211582, #101339, #177433, #191997, #110555, #97204, #204453, #70982, #128486, #256983, #84497, #55531, #168564, #36258, #32834 ) ) ;
#233085=VERTEX_POINT ( 'NONE', #16293 ) ;
#233344=FACE_OUTER_BOUND ( 'NONE', #125209, .T. ) ;
#233669=LINE ( 'NONE', #75867, #91036 ) ;
#233789=DIRECTION ( 'NONE',  ( 1.000000000000000000, 0.000000000000000000, 0.000000000000000000 ) ) ;
#233966=( NAMED_UNIT ( * ) SI_UNIT ( $, .STERADIAN. ) SOLID_ANGLE_UNIT ( ) );
#234853=DIRECTION ( 'NONE',  ( 0.000000000000000000, 0.000000000000000000, 1.000000000000000000 ) ) ;
#235434=CARTESIAN_POINT ( 'NONE',  ( -23.30000000000000426, -11.79999999999999893, 33.00000000000000000 ) ) ;
#235689=EDGE_CURVE ( 'NONE', #58739, #204353, #41767, .T. ) ;
#236555=CIRCLE ( 'NONE', #11741, 10.00000000000000178 ) ;
#237451=FACE_OUTER_BOUND ( 'NONE', #231386, .T. ) ;
#237761=VERTEX_POINT ( 'NONE', #127113 ) ;
#238087=PLANE ( 'NONE',  #101343 ) ;
#238314=DIRECTION ( 'NONE',  ( -1.000000000000000000, 0.000000000000000000, 0.000000000000000000 ) ) ;
#238317=DIRECTION ( 'NONE',  ( 0.000000000000000000, 0.000000000000000000, 1.000000000000000000 ) ) ;
#239025=FACE_OUTER_BOUND ( 'NONE', #157251, .T. ) ;
#239187=DIRECTION ( 'NONE',  ( -0.000000000000000000, 0.000000000000000000, -1.000000000000000000 ) ) ;
#239541=CARTESIAN_POINT ( 'NONE',  ( 27.30103769104855971, 12.20000000000000284, -347.0000000000001137 ) ) ;
#239615=CARTESIAN_POINT ( 'NONE',  ( -33.80000000000000426, 3.175288713399618601, -347.0000000000001137 ) ) ;
#239706=ORIENTED_EDGE ( 'NONE', *, *, #217458, .F. ) ;
#239779=CARTESIAN_POINT ( 'NONE',  ( -24.30000000000000071, 3.175288713399619933, 33.00000000000000000 ) ) ;
#239977=DIRECTION ( 'NONE',  ( 0.000000000000000000, 0.000000000000000000, 1.000000000000000000 ) ) ;
#240473=VECTOR ( 'NONE', #165524, 1000.000000000000000 ) ;
#240879=EDGE_LOOP ( 'NONE', ( #62381, #160515, #251251, #30300 ) ) ;
#242650=AXIS2_PLACEMENT_3D ( 'NONE', #18849, #239187, #157102 ) ;
#242707=FILL_AREA_STYLE_COLOUR ( '', #79246 ) ;
#243231=DIRECTION ( 'NONE',  ( -0.8191520442889921316, -0.5735764363510457153, 0.000000000000000000 ) ) ;
#244534=SURFACE_STYLE_FILL_AREA ( #85432 ) ;
#245445=VECTOR ( 'NONE', #223066, 1000.000000000000000 ) ;
#247353=ORIENTED_EDGE ( 'NONE', *, *, #229521, .F. ) ;
#248262=ORIENTED_EDGE ( 'NONE', *, *, #115777, .T. ) ;
#248426=DIRECTION ( 'NONE',  ( 0.000000000000000000, 0.000000000000000000, 1.000000000000000000 ) ) ;
#249548=DIRECTION ( 'NONE',  ( 0.8191520442889914655, 0.5735764363510466035, -0.000000000000000000 ) ) ;
#250001=ORIENTED_EDGE ( 'NONE', *, *, #21145, .F. ) ;
#250374=LINE ( 'NONE', #95153, #147146 ) ;
#250971=CARTESIAN_POINT ( 'NONE',  ( -23.30000000000000426, -11.79999999999999893, -347.0000000000001137 ) ) ;
#251251=ORIENTED_EDGE ( 'NONE', *, *, #253132, .T. ) ;
#251880=DIRECTION ( 'NONE',  ( 1.000000000000000000, 1.070816960479510500E-16, -0.000000000000000000 ) ) ;
#252060=ORIENTED_EDGE ( 'NONE', *, *, #6762, .F. ) ;
#252717=PLANE ( 'NONE',  #114332 ) ;
#252988=EDGE_CURVE ( 'NONE', #5597, #58739, #225222, .T. ) ;
#253132=EDGE_CURVE ( 'NONE', #66177, #170483, #139999, .T. ) ;
#254523=CARTESIAN_POINT ( 'NONE',  ( 24.30000000000000071, 3.175288713399624818, -347.0000000000001137 ) ) ;
#254748=CARTESIAN_POINT ( 'NONE',  ( -24.30000000000000071, -12.80000000000000249, -347.0000000000001137 ) ) ;
#254890=CARTESIAN_POINT ( 'NONE',  ( 24.30000000000000071, 3.175288713399624818, 33.00000000000000000 ) ) ;
#254973=LINE ( 'NONE', #197626, #29963 ) ;
#255096=ADVANCED_FACE ( 'NONE', ( #7916 ), #185253, .T. ) ;
#255593=ORIENTED_EDGE ( 'NONE', *, *, #212823, .T. ) ;
#255832=VECTOR ( 'NONE', #101111, 1000.000000000000000 ) ;
#256282=ORIENTED_EDGE ( 'NONE', *, *, #94230, .T. ) ;
#256914=PLANE ( 'NONE',  #186170 ) ;
#256983=ORIENTED_EDGE ( 'NONE', *, *, #34764, .F. ) ;
#257321=EDGE_CURVE ( 'NONE', #201551, #40973, #5882, .T. ) ;
#257517=DIRECTION ( 'NONE',  ( -1.000000000000000000, -1.116774769942150098E-16, -0.000000000000000000 ) ) ;
#257586=ADVANCED_FACE ( 'NONE', ( #221725 ), #104347, .F. ) ;
#257818=DIRECTION ( 'NONE',  ( 1.000000000000000000, 0.000000000000000000, -0.000000000000000000 ) ) ;
ENDSEC;
END-ISO-10303-21;
